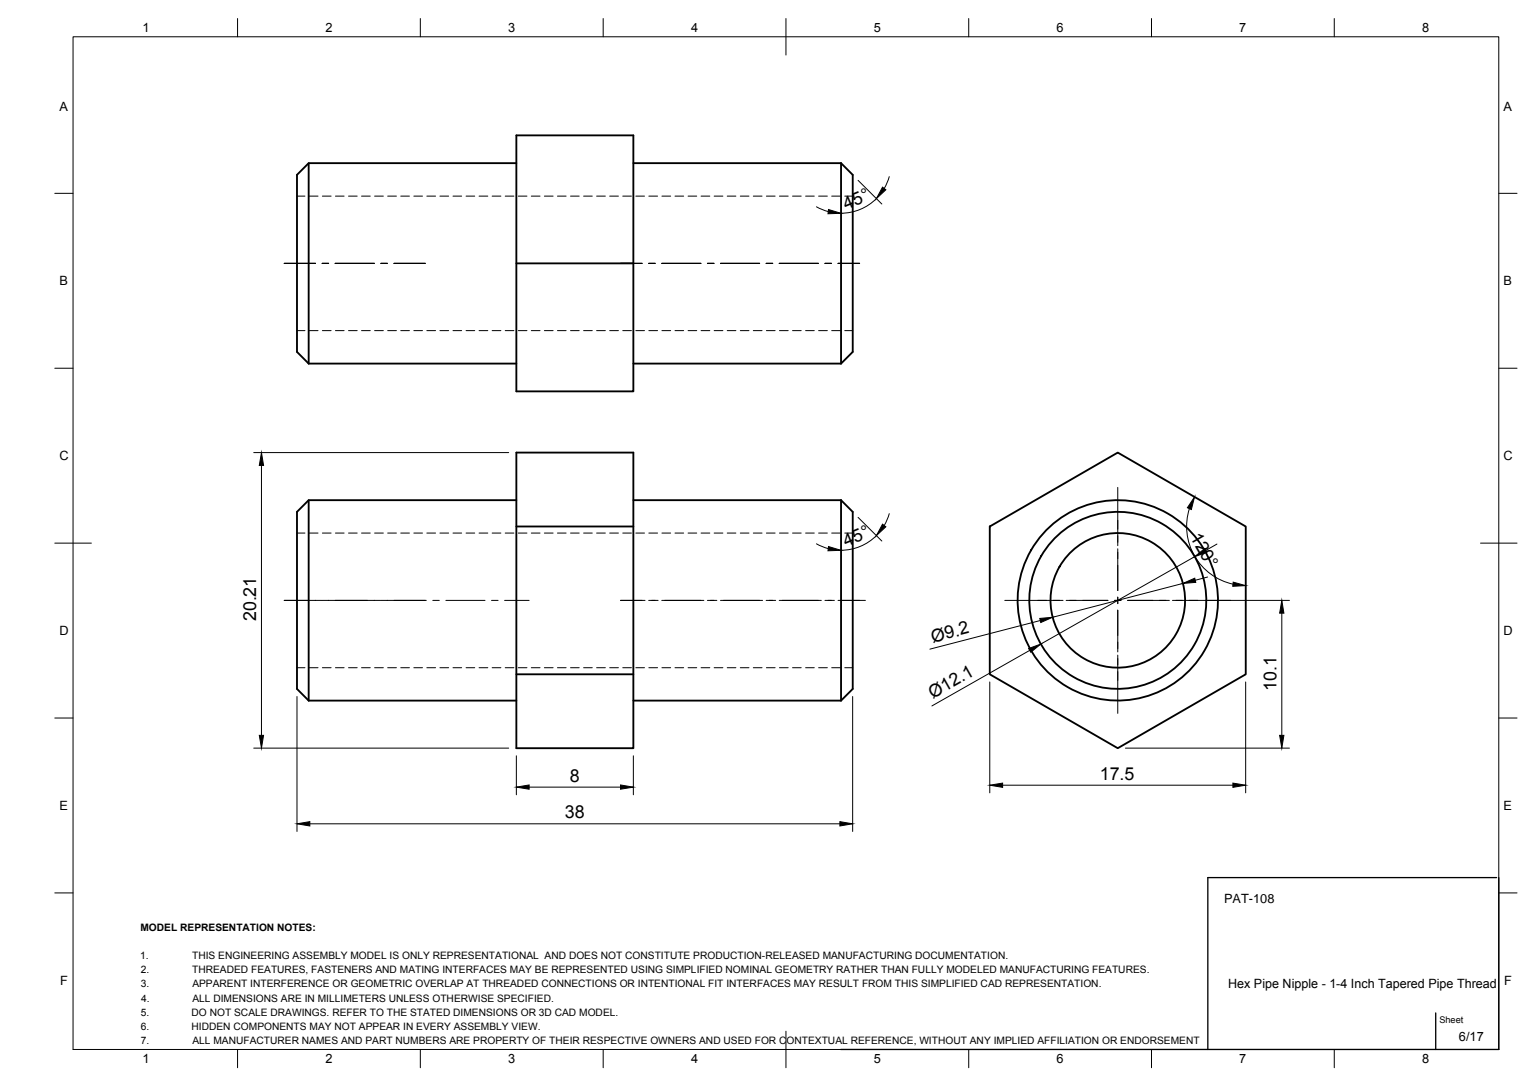
ISO-10303-21;
HEADER;
/* Generated by software containing ST-Developer
 * from STEP Tools, Inc. (www.steptools.com) 
 */

FILE_DESCRIPTION(
/* description */ ('Sub-base valve envelopes and connections'),
/* implementation_level */ '2;1');

FILE_NAME(
/* name */ 'Hex Pipe Nipple - 1-4 Inch Tapered Pipe Thread.step',
/* time_stamp */ '2026-10-29T15:55:44-07:00',
/* author */ (''),
/* organization */ (''),
/* preprocessor_version */ 'ST-DEVELOPER v20.2',
/* originating_system */ 'Autodesk Translation Framework v15.17.0.0',
/* authorisation */ '');

FILE_SCHEMA (('AUTOMOTIVE_DESIGN { 1 0 10303 214 3 1 1 }'));
ENDSEC;

DATA;
#10=MECHANICAL_DESIGN_GEOMETRIC_PRESENTATION_REPRESENTATION('',(#122),#6113);
#89=CONICAL_SURFACE('',#3689,0.645,0.785398163397448);
#90=CONICAL_SURFACE('',#3692,0.645,0.785398163397448);
#98=SHAPE_REPRESENTATION_RELATIONSHIP('SRR','None',#6171,#110);
#110=ADVANCED_BREP_SHAPE_REPRESENTATION('',(#134),#6102);
#122=STYLED_ITEM('',(#6308),#134);
#134=MANIFOLD_SOLID_BREP('Body1',#3361);
#206=FACE_BOUND('',#727,.T.);
#207=FACE_BOUND('',#729,.T.);
#208=FACE_BOUND('',#738,.T.);
#209=FACE_BOUND('',#743,.T.);
#307=PLANE('',#3674);
#308=PLANE('',#3676);
#309=PLANE('',#3678);
#310=PLANE('',#3679);
#311=PLANE('',#3680);
#312=PLANE('',#3681);
#313=PLANE('',#3682);
#314=PLANE('',#3683);
#315=PLANE('',#3686);
#316=PLANE('',#3694);
#463=FACE_OUTER_BOUND('',#726,.T.);
#464=FACE_OUTER_BOUND('',#728,.T.);
#465=FACE_OUTER_BOUND('',#730,.T.);
#466=FACE_OUTER_BOUND('',#731,.T.);
#467=FACE_OUTER_BOUND('',#732,.T.);
#468=FACE_OUTER_BOUND('',#733,.T.);
#469=FACE_OUTER_BOUND('',#734,.T.);
#470=FACE_OUTER_BOUND('',#735,.T.);
#471=FACE_OUTER_BOUND('',#736,.T.);
#472=FACE_OUTER_BOUND('',#737,.T.);
#473=FACE_OUTER_BOUND('',#739,.T.);
#474=FACE_OUTER_BOUND('',#740,.T.);
#475=FACE_OUTER_BOUND('',#741,.T.);
#476=FACE_OUTER_BOUND('',#742,.T.);
#477=FACE_OUTER_BOUND('',#744,.T.);
#726=EDGE_LOOP('',(#2577,#2578,#2579,#2580,#2581,#2582));
#727=EDGE_LOOP('',(#2583));
#728=EDGE_LOOP('',(#2584,#2585,#2586,#2587,#2588,#2589));
#729=EDGE_LOOP('',(#2590));
#730=EDGE_LOOP('',(#2591,#2592,#2593,#2594));
#731=EDGE_LOOP('',(#2595,#2596,#2597,#2598));
#732=EDGE_LOOP('',(#2599,#2600,#2601,#2602));
#733=EDGE_LOOP('',(#2603,#2604,#2605,#2606));
#734=EDGE_LOOP('',(#2607,#2608,#2609,#2610));
#735=EDGE_LOOP('',(#2611,#2612,#2613,#2614));
#736=EDGE_LOOP('',(#2615,#2616,#2617,#2618));
#737=EDGE_LOOP('',(#2619));
#738=EDGE_LOOP('',(#2620));
#739=EDGE_LOOP('',(#2621,#2622,#2623,#2624));
#740=EDGE_LOOP('',(#2625,#2626,#2627,#2628));
#741=EDGE_LOOP('',(#2629,#2630,#2631,#2632));
#742=EDGE_LOOP('',(#2633));
#743=EDGE_LOOP('',(#2634));
#744=EDGE_LOOP('',(#2635,#2636,#2637,#2638));
#966=LINE('',#5521,#1200);
#967=LINE('',#5523,#1201);
#968=LINE('',#5525,#1202);
#969=LINE('',#5527,#1203);
#970=LINE('',#5529,#1204);
#971=LINE('',#5530,#1205);
#972=LINE('',#5536,#1206);
#973=LINE('',#5538,#1207);
#974=LINE('',#5540,#1208);
#975=LINE('',#5542,#1209);
#976=LINE('',#5544,#1210);
#977=LINE('',#5545,#1211);
#978=LINE('',#5549,#1212);
#979=LINE('',#5550,#1213);
#980=LINE('',#5552,#1214);
#981=LINE('',#5554,#1215);
#982=LINE('',#5556,#1216);
#983=LINE('',#5558,#1217);
#984=LINE('',#5562,#1218);
#985=LINE('',#5570,#1219);
#986=LINE('',#5574,#1220);
#987=LINE('',#5578,#1221);
#988=LINE('',#5583,#1222);
#1200=VECTOR('',#4312,1.);
#1201=VECTOR('',#4313,1.);
#1202=VECTOR('',#4314,1.);
#1203=VECTOR('',#4315,1.);
#1204=VECTOR('',#4316,1.);
#1205=VECTOR('',#4317,1.);
#1206=VECTOR('',#4322,1.);
#1207=VECTOR('',#4323,1.);
#1208=VECTOR('',#4324,1.);
#1209=VECTOR('',#4325,1.);
#1210=VECTOR('',#4326,1.);
#1211=VECTOR('',#4327,1.);
#1212=VECTOR('',#4332,1.);
#1213=VECTOR('',#4333,1.);
#1214=VECTOR('',#4336,1.);
#1215=VECTOR('',#4339,1.);
#1216=VECTOR('',#4342,1.);
#1217=VECTOR('',#4345,1.);
#1218=VECTOR('',#4350,0.685);
#1219=VECTOR('',#4361,0.645);
#1220=VECTOR('',#4366,0.685);
#1221=VECTOR('',#4371,0.645);
#1222=VECTOR('',#4378,0.46);
#1457=CIRCLE('',#3675,0.685);
#1458=CIRCLE('',#3677,0.685);
#1459=CIRCLE('',#3685,0.685);
#1460=CIRCLE('',#3687,0.605);
#1461=CIRCLE('',#3688,0.46);
#1462=CIRCLE('',#3691,0.685);
#1463=CIRCLE('',#3693,0.605);
#1464=CIRCLE('',#3695,0.46);
#1651=VERTEX_POINT('',#5519);
#1652=VERTEX_POINT('',#5520);
#1653=VERTEX_POINT('',#5522);
#1654=VERTEX_POINT('',#5524);
#1655=VERTEX_POINT('',#5526);
#1656=VERTEX_POINT('',#5528);
#1657=VERTEX_POINT('',#5531);
#1658=VERTEX_POINT('',#5534);
#1659=VERTEX_POINT('',#5535);
#1660=VERTEX_POINT('',#5537);
#1661=VERTEX_POINT('',#5539);
#1662=VERTEX_POINT('',#5541);
#1663=VERTEX_POINT('',#5543);
#1664=VERTEX_POINT('',#5546);
#1665=VERTEX_POINT('',#5561);
#1666=VERTEX_POINT('',#5565);
#1667=VERTEX_POINT('',#5567);
#1668=VERTEX_POINT('',#5572);
#1669=VERTEX_POINT('',#5576);
#1670=VERTEX_POINT('',#5580);
#1986=EDGE_CURVE('',#1651,#1652,#966,.T.);
#1987=EDGE_CURVE('',#1652,#1653,#967,.T.);
#1988=EDGE_CURVE('',#1653,#1654,#968,.T.);
#1989=EDGE_CURVE('',#1654,#1655,#969,.T.);
#1990=EDGE_CURVE('',#1655,#1656,#970,.T.);
#1991=EDGE_CURVE('',#1656,#1651,#971,.T.);
#1992=EDGE_CURVE('',#1657,#1657,#1457,.T.);
#1993=EDGE_CURVE('',#1658,#1659,#972,.T.);
#1994=EDGE_CURVE('',#1659,#1660,#973,.T.);
#1995=EDGE_CURVE('',#1660,#1661,#974,.T.);
#1996=EDGE_CURVE('',#1661,#1662,#975,.T.);
#1997=EDGE_CURVE('',#1662,#1663,#976,.T.);
#1998=EDGE_CURVE('',#1663,#1658,#977,.T.);
#1999=EDGE_CURVE('',#1664,#1664,#1458,.T.);
#2000=EDGE_CURVE('',#1658,#1652,#978,.T.);
#2001=EDGE_CURVE('',#1653,#1663,#979,.T.);
#2002=EDGE_CURVE('',#1654,#1662,#980,.T.);
#2003=EDGE_CURVE('',#1655,#1661,#981,.T.);
#2004=EDGE_CURVE('',#1656,#1660,#982,.T.);
#2005=EDGE_CURVE('',#1651,#1659,#983,.T.);
#2006=EDGE_CURVE('',#1664,#1665,#984,.T.);
#2007=EDGE_CURVE('',#1665,#1665,#1459,.T.);
#2008=EDGE_CURVE('',#1666,#1666,#1460,.T.);
#2009=EDGE_CURVE('',#1667,#1667,#1461,.T.);
#2010=EDGE_CURVE('',#1665,#1666,#985,.T.);
#2011=EDGE_CURVE('',#1668,#1668,#1462,.T.);
#2012=EDGE_CURVE('',#1668,#1657,#986,.T.);
#2013=EDGE_CURVE('',#1669,#1669,#1463,.T.);
#2014=EDGE_CURVE('',#1669,#1668,#987,.T.);
#2015=EDGE_CURVE('',#1670,#1670,#1464,.T.);
#2016=EDGE_CURVE('',#1670,#1667,#988,.T.);
#2577=ORIENTED_EDGE('',*,*,#1986,.T.);
#2578=ORIENTED_EDGE('',*,*,#1987,.T.);
#2579=ORIENTED_EDGE('',*,*,#1988,.T.);
#2580=ORIENTED_EDGE('',*,*,#1989,.T.);
#2581=ORIENTED_EDGE('',*,*,#1990,.T.);
#2582=ORIENTED_EDGE('',*,*,#1991,.T.);
#2583=ORIENTED_EDGE('',*,*,#1992,.F.);
#2584=ORIENTED_EDGE('',*,*,#1993,.T.);
#2585=ORIENTED_EDGE('',*,*,#1994,.T.);
#2586=ORIENTED_EDGE('',*,*,#1995,.T.);
#2587=ORIENTED_EDGE('',*,*,#1996,.T.);
#2588=ORIENTED_EDGE('',*,*,#1997,.T.);
#2589=ORIENTED_EDGE('',*,*,#1998,.T.);
#2590=ORIENTED_EDGE('',*,*,#1999,.F.);
#2591=ORIENTED_EDGE('',*,*,#2000,.F.);
#2592=ORIENTED_EDGE('',*,*,#1998,.F.);
#2593=ORIENTED_EDGE('',*,*,#2001,.F.);
#2594=ORIENTED_EDGE('',*,*,#1987,.F.);
#2595=ORIENTED_EDGE('',*,*,#2001,.T.);
#2596=ORIENTED_EDGE('',*,*,#1997,.F.);
#2597=ORIENTED_EDGE('',*,*,#2002,.F.);
#2598=ORIENTED_EDGE('',*,*,#1988,.F.);
#2599=ORIENTED_EDGE('',*,*,#2002,.T.);
#2600=ORIENTED_EDGE('',*,*,#1996,.F.);
#2601=ORIENTED_EDGE('',*,*,#2003,.F.);
#2602=ORIENTED_EDGE('',*,*,#1989,.F.);
#2603=ORIENTED_EDGE('',*,*,#2003,.T.);
#2604=ORIENTED_EDGE('',*,*,#1995,.F.);
#2605=ORIENTED_EDGE('',*,*,#2004,.F.);
#2606=ORIENTED_EDGE('',*,*,#1990,.F.);
#2607=ORIENTED_EDGE('',*,*,#2004,.T.);
#2608=ORIENTED_EDGE('',*,*,#1994,.F.);
#2609=ORIENTED_EDGE('',*,*,#2005,.F.);
#2610=ORIENTED_EDGE('',*,*,#1991,.F.);
#2611=ORIENTED_EDGE('',*,*,#2005,.T.);
#2612=ORIENTED_EDGE('',*,*,#1993,.F.);
#2613=ORIENTED_EDGE('',*,*,#2000,.T.);
#2614=ORIENTED_EDGE('',*,*,#1986,.F.);
#2615=ORIENTED_EDGE('',*,*,#1999,.T.);
#2616=ORIENTED_EDGE('',*,*,#2006,.T.);
#2617=ORIENTED_EDGE('',*,*,#2007,.T.);
#2618=ORIENTED_EDGE('',*,*,#2006,.F.);
#2619=ORIENTED_EDGE('',*,*,#2008,.F.);
#2620=ORIENTED_EDGE('',*,*,#2009,.T.);
#2621=ORIENTED_EDGE('',*,*,#2007,.F.);
#2622=ORIENTED_EDGE('',*,*,#2010,.T.);
#2623=ORIENTED_EDGE('',*,*,#2008,.T.);
#2624=ORIENTED_EDGE('',*,*,#2010,.F.);
#2625=ORIENTED_EDGE('',*,*,#2011,.F.);
#2626=ORIENTED_EDGE('',*,*,#2012,.T.);
#2627=ORIENTED_EDGE('',*,*,#1992,.T.);
#2628=ORIENTED_EDGE('',*,*,#2012,.F.);
#2629=ORIENTED_EDGE('',*,*,#2013,.F.);
#2630=ORIENTED_EDGE('',*,*,#2014,.T.);
#2631=ORIENTED_EDGE('',*,*,#2011,.T.);
#2632=ORIENTED_EDGE('',*,*,#2014,.F.);
#2633=ORIENTED_EDGE('',*,*,#2013,.T.);
#2634=ORIENTED_EDGE('',*,*,#2015,.F.);
#2635=ORIENTED_EDGE('',*,*,#2015,.T.);
#2636=ORIENTED_EDGE('',*,*,#2016,.T.);
#2637=ORIENTED_EDGE('',*,*,#2009,.F.);
#2638=ORIENTED_EDGE('',*,*,#2016,.F.);
#3122=CYLINDRICAL_SURFACE('',#3684,0.685);
#3123=CYLINDRICAL_SURFACE('',#3690,0.685);
#3124=CYLINDRICAL_SURFACE('',#3696,0.46);
#3236=ADVANCED_FACE('',(#463,#206),#307,.F.);
#3237=ADVANCED_FACE('',(#464,#207),#308,.T.);
#3238=ADVANCED_FACE('',(#465),#309,.T.);
#3239=ADVANCED_FACE('',(#466),#310,.T.);
#3240=ADVANCED_FACE('',(#467),#311,.T.);
#3241=ADVANCED_FACE('',(#468),#312,.T.);
#3242=ADVANCED_FACE('',(#469),#313,.T.);
#3243=ADVANCED_FACE('',(#470),#314,.T.);
#3244=ADVANCED_FACE('',(#471),#3122,.T.);
#3245=ADVANCED_FACE('',(#472,#208),#315,.T.);
#3246=ADVANCED_FACE('',(#473),#89,.T.);
#3247=ADVANCED_FACE('',(#474),#3123,.T.);
#3248=ADVANCED_FACE('',(#475),#90,.T.);
#3249=ADVANCED_FACE('',(#476,#209),#316,.T.);
#3250=ADVANCED_FACE('',(#477),#3124,.F.);
#3361=CLOSED_SHELL('',(#3236,#3237,#3238,#3239,#3240,#3241,#3242,#3243,
#3244,#3245,#3246,#3247,#3248,#3249,#3250));
#3673=AXIS2_PLACEMENT_3D('',#5517,#4308,#4309);
#3674=AXIS2_PLACEMENT_3D('',#5518,#4310,#4311);
#3675=AXIS2_PLACEMENT_3D('',#5532,#4318,#4319);
#3676=AXIS2_PLACEMENT_3D('',#5533,#4320,#4321);
#3677=AXIS2_PLACEMENT_3D('',#5547,#4328,#4329);
#3678=AXIS2_PLACEMENT_3D('',#5548,#4330,#4331);
#3679=AXIS2_PLACEMENT_3D('',#5551,#4334,#4335);
#3680=AXIS2_PLACEMENT_3D('',#5553,#4337,#4338);
#3681=AXIS2_PLACEMENT_3D('',#5555,#4340,#4341);
#3682=AXIS2_PLACEMENT_3D('',#5557,#4343,#4344);
#3683=AXIS2_PLACEMENT_3D('',#5559,#4346,#4347);
#3684=AXIS2_PLACEMENT_3D('',#5560,#4348,#4349);
#3685=AXIS2_PLACEMENT_3D('',#5563,#4351,#4352);
#3686=AXIS2_PLACEMENT_3D('',#5564,#4353,#4354);
#3687=AXIS2_PLACEMENT_3D('',#5566,#4355,#4356);
#3688=AXIS2_PLACEMENT_3D('',#5568,#4357,#4358);
#3689=AXIS2_PLACEMENT_3D('',#5569,#4359,#4360);
#3690=AXIS2_PLACEMENT_3D('',#5571,#4362,#4363);
#3691=AXIS2_PLACEMENT_3D('',#5573,#4364,#4365);
#3692=AXIS2_PLACEMENT_3D('',#5575,#4367,#4368);
#3693=AXIS2_PLACEMENT_3D('',#5577,#4369,#4370);
#3694=AXIS2_PLACEMENT_3D('',#5579,#4372,#4373);
#3695=AXIS2_PLACEMENT_3D('',#5581,#4374,#4375);
#3696=AXIS2_PLACEMENT_3D('',#5582,#4376,#4377);
#4308=DIRECTION('axis',(0.,0.,1.));
#4309=DIRECTION('refdir',(1.,0.,0.));
#4310=DIRECTION('center_axis',(0.,1.,0.));
#4311=DIRECTION('ref_axis',(1.,0.,0.));
#4312=DIRECTION('',(-0.5,0.,0.866025403784439));
#4313=DIRECTION('',(-1.,0.,-3.29650746237182E-16));
#4314=DIRECTION('',(-0.5,0.,-0.866025403784439));
#4315=DIRECTION('',(0.5,0.,-0.866025403784438));
#4316=DIRECTION('',(1.,0.,0.));
#4317=DIRECTION('',(0.5,0.,0.866025403784439));
#4318=DIRECTION('center_axis',(0.,-1.,0.));
#4319=DIRECTION('ref_axis',(1.,0.,0.));
#4320=DIRECTION('center_axis',(0.,1.,0.));
#4321=DIRECTION('ref_axis',(1.,0.,0.));
#4322=DIRECTION('',(0.5,0.,-0.866025403784439));
#4323=DIRECTION('',(-0.5,0.,-0.866025403784439));
#4324=DIRECTION('',(-1.,0.,0.));
#4325=DIRECTION('',(-0.5,0.,0.866025403784438));
#4326=DIRECTION('',(0.5,0.,0.866025403784439));
#4327=DIRECTION('',(1.,0.,3.29650746237182E-16));
#4328=DIRECTION('center_axis',(0.,1.,0.));
#4329=DIRECTION('ref_axis',(1.,0.,0.));
#4330=DIRECTION('center_axis',(-3.29650746237182E-16,0.,1.));
#4331=DIRECTION('ref_axis',(1.,0.,3.29650746237182E-16));
#4332=DIRECTION('',(0.,-1.,0.));
#4333=DIRECTION('',(0.,1.,0.));
#4334=DIRECTION('center_axis',(-0.866025403784439,0.,0.5));
#4335=DIRECTION('ref_axis',(0.5,0.,0.866025403784439));
#4336=DIRECTION('',(0.,1.,0.));
#4337=DIRECTION('center_axis',(-0.866025403784439,0.,-0.5));
#4338=DIRECTION('ref_axis',(-0.5,0.,0.866025403784439));
#4339=DIRECTION('',(0.,1.,0.));
#4340=DIRECTION('center_axis',(0.,0.,-1.));
#4341=DIRECTION('ref_axis',(-1.,0.,0.));
#4342=DIRECTION('',(0.,1.,0.));
#4343=DIRECTION('center_axis',(0.866025403784439,0.,-0.5));
#4344=DIRECTION('ref_axis',(-0.5,0.,-0.866025403784439));
#4345=DIRECTION('',(0.,1.,0.));
#4346=DIRECTION('center_axis',(0.866025403784439,0.,0.5));
#4347=DIRECTION('ref_axis',(0.5,0.,-0.866025403784439));
#4348=DIRECTION('center_axis',(0.,-1.,0.));
#4349=DIRECTION('ref_axis',(1.,0.,0.));
#4350=DIRECTION('',(0.,1.,0.));
#4351=DIRECTION('center_axis',(0.,-1.,0.));
#4352=DIRECTION('ref_axis',(1.,0.,0.));
#4353=DIRECTION('center_axis',(0.,1.,0.));
#4354=DIRECTION('ref_axis',(0.,0.,1.));
#4355=DIRECTION('center_axis',(0.,-1.,0.));
#4356=DIRECTION('ref_axis',(1.,0.,0.));
#4357=DIRECTION('center_axis',(0.,-1.,0.));
#4358=DIRECTION('ref_axis',(1.,0.,0.));
#4359=DIRECTION('center_axis',(0.,-1.,0.));
#4360=DIRECTION('ref_axis',(1.,0.,0.));
#4361=DIRECTION('',(0.707106781186547,0.707106781186548,8.65956056235493E-17));
#4362=DIRECTION('center_axis',(0.,-1.,0.));
#4363=DIRECTION('ref_axis',(1.,0.,0.));
#4364=DIRECTION('center_axis',(0.,-1.,0.));
#4365=DIRECTION('ref_axis',(1.,0.,0.));
#4366=DIRECTION('',(0.,1.,0.));
#4367=DIRECTION('center_axis',(0.,1.,0.));
#4368=DIRECTION('ref_axis',(1.,0.,0.));
#4369=DIRECTION('center_axis',(0.,-1.,0.));
#4370=DIRECTION('ref_axis',(1.,0.,0.));
#4371=DIRECTION('',(-0.707106781186547,0.707106781186548,-8.65956056235493E-17));
#4372=DIRECTION('center_axis',(0.,-1.,0.));
#4373=DIRECTION('ref_axis',(0.,0.,-1.));
#4374=DIRECTION('center_axis',(0.,-1.,0.));
#4375=DIRECTION('ref_axis',(1.,0.,0.));
#4376=DIRECTION('center_axis',(0.,-1.,0.));
#4377=DIRECTION('ref_axis',(1.,0.,0.));
#4378=DIRECTION('',(0.,1.,0.));
#5517=CARTESIAN_POINT('',(0.,0.,0.));
#5518=CARTESIAN_POINT('Origin',(0.,-0.4,0.));
#5519=CARTESIAN_POINT('',(1.01036297108185,-0.4,0.));
#5520=CARTESIAN_POINT('',(0.505181485540923,-0.4,0.875));
#5521=CARTESIAN_POINT('',(0.505181485540923,-0.4,0.875));
#5522=CARTESIAN_POINT('',(-0.505181485540923,-0.4,0.875));
#5523=CARTESIAN_POINT('',(-0.505181485540923,-0.4,0.875));
#5524=CARTESIAN_POINT('',(-1.01036297108185,-0.4,-1.23733777851239E-16));
#5525=CARTESIAN_POINT('',(-1.01036297108185,-0.4,-1.23733777851239E-16));
#5526=CARTESIAN_POINT('',(-0.505181485540922,-0.4,-0.875));
#5527=CARTESIAN_POINT('',(-0.505181485540922,-0.4,-0.875));
#5528=CARTESIAN_POINT('',(0.505181485540923,-0.4,-0.875));
#5529=CARTESIAN_POINT('',(0.505181485540923,-0.4,-0.875));
#5530=CARTESIAN_POINT('',(1.01036297108185,-0.4,0.));
#5531=CARTESIAN_POINT('',(-0.685,-0.4,-8.38883057415937E-17));
#5532=CARTESIAN_POINT('Origin',(0.,-0.4,0.));
#5533=CARTESIAN_POINT('Origin',(0.,0.4,0.));
#5534=CARTESIAN_POINT('',(0.505181485540923,0.4,0.875));
#5535=CARTESIAN_POINT('',(1.01036297108185,0.4,0.));
#5536=CARTESIAN_POINT('',(0.505181485540923,0.4,0.875));
#5537=CARTESIAN_POINT('',(0.505181485540923,0.4,-0.875));
#5538=CARTESIAN_POINT('',(1.01036297108185,0.4,0.));
#5539=CARTESIAN_POINT('',(-0.505181485540922,0.4,-0.875));
#5540=CARTESIAN_POINT('',(0.505181485540923,0.4,-0.875));
#5541=CARTESIAN_POINT('',(-1.01036297108185,0.4,-1.23733777851239E-16));
#5542=CARTESIAN_POINT('',(-0.505181485540922,0.4,-0.875));
#5543=CARTESIAN_POINT('',(-0.505181485540923,0.4,0.875));
#5544=CARTESIAN_POINT('',(-1.01036297108185,0.4,-1.23733777851239E-16));
#5545=CARTESIAN_POINT('',(-0.505181485540923,0.4,0.875));
#5546=CARTESIAN_POINT('',(-0.685,0.4,8.38883057415937E-17));
#5547=CARTESIAN_POINT('Origin',(0.,0.4,0.));
#5548=CARTESIAN_POINT('Origin',(-0.505181485540923,0.,0.875));
#5549=CARTESIAN_POINT('',(0.505181485540923,0.,0.875));
#5550=CARTESIAN_POINT('',(-0.505181485540923,0.,0.875));
#5551=CARTESIAN_POINT('Origin',(-1.01036297108185,0.,-1.23733777851239E-16));
#5552=CARTESIAN_POINT('',(-1.01036297108185,0.,-1.23733777851239E-16));
#5553=CARTESIAN_POINT('Origin',(-0.505181485540922,0.,-0.875));
#5554=CARTESIAN_POINT('',(-0.505181485540922,0.,-0.875));
#5555=CARTESIAN_POINT('Origin',(0.505181485540923,0.,-0.875));
#5556=CARTESIAN_POINT('',(0.505181485540923,0.,-0.875));
#5557=CARTESIAN_POINT('Origin',(1.01036297108185,0.,0.));
#5558=CARTESIAN_POINT('',(1.01036297108185,0.,0.));
#5559=CARTESIAN_POINT('Origin',(0.505181485540923,0.,0.875));
#5560=CARTESIAN_POINT('Origin',(0.,0.,0.));
#5561=CARTESIAN_POINT('',(-0.685,1.82,-8.38883057415937E-17));
#5562=CARTESIAN_POINT('',(-0.685,0.,-8.38883057415937E-17));
#5563=CARTESIAN_POINT('Origin',(0.,1.82,0.));
#5564=CARTESIAN_POINT('Origin',(0.605,1.9,0.));
#5565=CARTESIAN_POINT('',(-0.605,1.9,-7.40911313484149E-17));
#5566=CARTESIAN_POINT('Origin',(0.,1.9,0.));
#5567=CARTESIAN_POINT('',(-0.46,1.9,-5.63337527607782E-17));
#5568=CARTESIAN_POINT('Origin',(0.,1.9,0.));
#5569=CARTESIAN_POINT('Origin',(0.,1.86,0.));
#5570=CARTESIAN_POINT('',(-0.645,1.86,-7.89897185450043E-17));
#5571=CARTESIAN_POINT('Origin',(0.,0.,0.));
#5572=CARTESIAN_POINT('',(-0.685,-1.82,-8.38883057415937E-17));
#5573=CARTESIAN_POINT('Origin',(0.,-1.82,0.));
#5574=CARTESIAN_POINT('',(-0.685,0.,-8.38883057415937E-17));
#5575=CARTESIAN_POINT('Origin',(0.,-1.86,0.));
#5576=CARTESIAN_POINT('',(-0.605,-1.9,-7.40911313484149E-17));
#5577=CARTESIAN_POINT('Origin',(0.,-1.9,0.));
#5578=CARTESIAN_POINT('',(-0.645,-1.86,-7.89897185450043E-17));
#5579=CARTESIAN_POINT('Origin',(0.46,-1.9,0.));
#5580=CARTESIAN_POINT('',(-0.46,-1.9,-5.63337527607782E-17));
#5581=CARTESIAN_POINT('Origin',(0.,-1.9,0.));
#5582=CARTESIAN_POINT('Origin',(0.,0.,0.));
#5583=CARTESIAN_POINT('',(-0.46,0.,-5.63337527607782E-17));
#6086=UNCERTAINTY_MEASURE_WITH_UNIT(LENGTH_MEASURE(0.001),#6114,
'DISTANCE_ACCURACY_VALUE',
'Maximum model space distance between geometric entities at asserted c
onnectivities');
#6097=UNCERTAINTY_MEASURE_WITH_UNIT(LENGTH_MEASURE(0.001),#6114,
'DISTANCE_ACCURACY_VALUE',
'Maximum model space distance between geometric entities at asserted c
onnectivities');
#6102=(
GEOMETRIC_REPRESENTATION_CONTEXT(3)
GLOBAL_UNCERTAINTY_ASSIGNED_CONTEXT((#6086))
GLOBAL_UNIT_ASSIGNED_CONTEXT((#6114,#6116,#6117))
REPRESENTATION_CONTEXT('','3D')
);
#6113=(
GEOMETRIC_REPRESENTATION_CONTEXT(3)
GLOBAL_UNCERTAINTY_ASSIGNED_CONTEXT((#6097))
GLOBAL_UNIT_ASSIGNED_CONTEXT((#6114,#6116,#6117))
REPRESENTATION_CONTEXT('','3D')
);
#6114=(
LENGTH_UNIT()
NAMED_UNIT(*)
SI_UNIT(.CENTI.,.METRE.)
);
#6116=(
NAMED_UNIT(*)
PLANE_ANGLE_UNIT()
SI_UNIT($,.RADIAN.)
);
#6117=(
NAMED_UNIT(*)
SI_UNIT($,.STERADIAN.)
SOLID_ANGLE_UNIT()
);
#6122=SHAPE_DEFINITION_REPRESENTATION(#6137,#6171);
#6137=PRODUCT_DEFINITION_SHAPE('',$,#6187);
#6171=SHAPE_REPRESENTATION('',(#3673),#6102);
#6182=PRODUCT_DEFINITION_CONTEXT('part definition',#6229,'design');
#6187=PRODUCT_DEFINITION('Hex Pipe Nipple - 1-4 Inch Tapered Pipe Thread',
'Hex Pipe Nipple - 1-4 Inch Tapered Pipe Thread',#6202,#6182);
#6202=PRODUCT_DEFINITION_FORMATION('',$,#6235);
#6229=APPLICATION_CONTEXT(
'Core Data for Automotive Mechanical Design Process');
#6230=PRODUCT_CONTEXT('part definition',#6229,'mechanical');
#6235=PRODUCT('Hex Pipe Nipple - 1-4 Inch Tapered Pipe Thread',
'Hex Pipe Nipple - 1-4 Inch Tapered Pipe Thread',
'Hex Pipe Nipple - 1-4 Inch Tapered Pipe Thread',(#6230));
#6302=COLOUR_RGB('Sky Blue',0.24,0.69,0.87);
#6303=FILL_AREA_STYLE_COLOUR('',#6302);
#6304=FILL_AREA_STYLE('',(#6303));
#6305=SURFACE_STYLE_FILL_AREA(#6304);
#6306=SURFACE_SIDE_STYLE('',(#6305));
#6307=SURFACE_STYLE_USAGE(.BOTH.,#6306);
#6308=PRESENTATION_STYLE_ASSIGNMENT((#6307));
ENDSEC;
END-ISO-10303-21;
